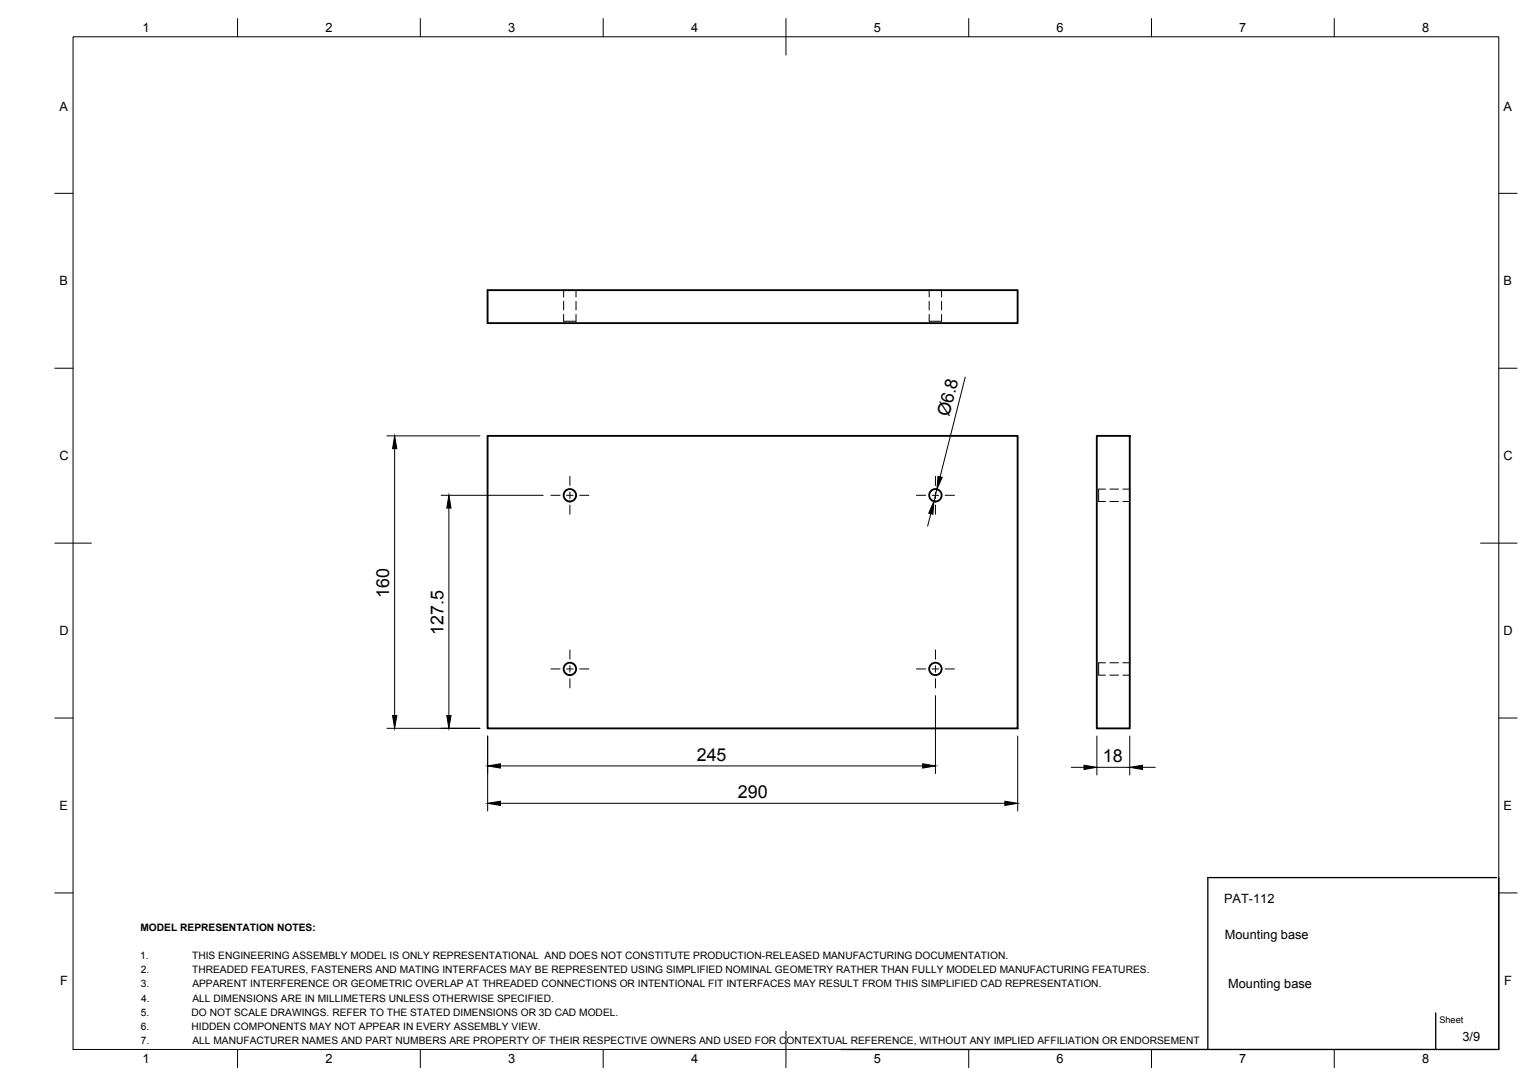
ISO-10303-21;
HEADER;
/* Generated by software containing ST-Developer
 * from STEP Tools, Inc. (www.steptools.com) 
 */

FILE_DESCRIPTION(
/* description */ ('PAT-112'),
/* implementation_level */ '2;1');

FILE_NAME(
/* name */ 'Mounting base.step',
/* time_stamp */ '2026-11-15T15:25:42-08:00',
/* author */ (''),
/* organization */ (''),
/* preprocessor_version */ 'ST-DEVELOPER v20.2',
/* originating_system */ 'Autodesk Translation Framework v15.17.0.0',
/* authorisation */ '');

FILE_SCHEMA (('AUTOMOTIVE_DESIGN { 1 0 10303 214 3 1 1 }'));
ENDSEC;

DATA;
#10=MECHANICAL_DESIGN_GEOMETRIC_PRESENTATION_REPRESENTATION('',(#105),#2277);
#91=SHAPE_REPRESENTATION_RELATIONSHIP('SRR','None',#2319,#98);
#98=ADVANCED_BREP_SHAPE_REPRESENTATION('',(#113),#2269);
#105=STYLED_ITEM('',(#2368),#113);
#113=MANIFOLD_SOLID_BREP('Body1',#1257);
#120=FACE_BOUND('',#287,.T.);
#121=FACE_BOUND('',#288,.T.);
#122=FACE_BOUND('',#289,.T.);
#123=FACE_BOUND('',#290,.T.);
#146=PLANE('',#1349);
#147=PLANE('',#1353);
#148=PLANE('',#1357);
#149=PLANE('',#1361);
#150=PLANE('',#1362);
#151=PLANE('',#1363);
#152=PLANE('',#1364);
#153=PLANE('',#1365);
#154=PLANE('',#1366);
#155=PLANE('',#1367);
#197=FACE_OUTER_BOUND('',#274,.T.);
#198=FACE_OUTER_BOUND('',#275,.T.);
#199=FACE_OUTER_BOUND('',#276,.T.);
#200=FACE_OUTER_BOUND('',#277,.T.);
#201=FACE_OUTER_BOUND('',#278,.T.);
#202=FACE_OUTER_BOUND('',#279,.T.);
#203=FACE_OUTER_BOUND('',#280,.T.);
#204=FACE_OUTER_BOUND('',#281,.T.);
#205=FACE_OUTER_BOUND('',#282,.T.);
#206=FACE_OUTER_BOUND('',#283,.T.);
#207=FACE_OUTER_BOUND('',#284,.T.);
#208=FACE_OUTER_BOUND('',#285,.T.);
#209=FACE_OUTER_BOUND('',#286,.T.);
#210=FACE_OUTER_BOUND('',#291,.T.);
#274=EDGE_LOOP('',(#866,#867,#868,#869));
#275=EDGE_LOOP('',(#870));
#276=EDGE_LOOP('',(#871,#872,#873,#874));
#277=EDGE_LOOP('',(#875));
#278=EDGE_LOOP('',(#876,#877,#878,#879));
#279=EDGE_LOOP('',(#880));
#280=EDGE_LOOP('',(#881,#882,#883,#884));
#281=EDGE_LOOP('',(#885));
#282=EDGE_LOOP('',(#886,#887,#888,#889));
#283=EDGE_LOOP('',(#890,#891,#892,#893));
#284=EDGE_LOOP('',(#894,#895,#896,#897));
#285=EDGE_LOOP('',(#898,#899,#900,#901));
#286=EDGE_LOOP('',(#902,#903,#904,#905));
#287=EDGE_LOOP('',(#906));
#288=EDGE_LOOP('',(#907));
#289=EDGE_LOOP('',(#908));
#290=EDGE_LOOP('',(#909));
#291=EDGE_LOOP('',(#910,#911,#912,#913));
#377=LINE('',#1913,#472);
#378=LINE('',#1920,#473);
#379=LINE('',#1927,#474);
#380=LINE('',#1934,#475);
#381=LINE('',#1940,#476);
#382=LINE('',#1942,#477);
#383=LINE('',#1944,#478);
#384=LINE('',#1945,#479);
#385=LINE('',#1948,#480);
#386=LINE('',#1950,#481);
#387=LINE('',#1951,#482);
#388=LINE('',#1954,#483);
#389=LINE('',#1956,#484);
#390=LINE('',#1957,#485);
#391=LINE('',#1959,#486);
#392=LINE('',#1960,#487);
#472=VECTOR('',#1508,0.34);
#473=VECTOR('',#1517,0.34);
#474=VECTOR('',#1526,0.34);
#475=VECTOR('',#1535,0.34);
#476=VECTOR('',#1542,1.);
#477=VECTOR('',#1543,1.);
#478=VECTOR('',#1544,1.);
#479=VECTOR('',#1545,1.);
#480=VECTOR('',#1548,1.);
#481=VECTOR('',#1549,1.);
#482=VECTOR('',#1550,1.);
#483=VECTOR('',#1553,1.);
#484=VECTOR('',#1554,1.);
#485=VECTOR('',#1555,1.);
#486=VECTOR('',#1558,1.);
#487=VECTOR('',#1559,1.);
#567=CIRCLE('',#1347,0.34);
#568=CIRCLE('',#1348,0.34);
#569=CIRCLE('',#1351,0.34);
#570=CIRCLE('',#1352,0.34);
#571=CIRCLE('',#1355,0.34);
#572=CIRCLE('',#1356,0.34);
#573=CIRCLE('',#1359,0.34);
#574=CIRCLE('',#1360,0.34);
#619=VERTEX_POINT('',#1910);
#620=VERTEX_POINT('',#1912);
#621=VERTEX_POINT('',#1917);
#622=VERTEX_POINT('',#1919);
#623=VERTEX_POINT('',#1924);
#624=VERTEX_POINT('',#1926);
#625=VERTEX_POINT('',#1931);
#626=VERTEX_POINT('',#1933);
#627=VERTEX_POINT('',#1938);
#628=VERTEX_POINT('',#1939);
#629=VERTEX_POINT('',#1941);
#630=VERTEX_POINT('',#1943);
#631=VERTEX_POINT('',#1947);
#632=VERTEX_POINT('',#1949);
#633=VERTEX_POINT('',#1953);
#634=VERTEX_POINT('',#1955);
#719=EDGE_CURVE('',#619,#619,#567,.T.);
#720=EDGE_CURVE('',#619,#620,#377,.T.);
#721=EDGE_CURVE('',#620,#620,#568,.T.);
#722=EDGE_CURVE('',#621,#621,#569,.T.);
#723=EDGE_CURVE('',#621,#622,#378,.T.);
#724=EDGE_CURVE('',#622,#622,#570,.T.);
#725=EDGE_CURVE('',#623,#623,#571,.T.);
#726=EDGE_CURVE('',#623,#624,#379,.T.);
#727=EDGE_CURVE('',#624,#624,#572,.T.);
#728=EDGE_CURVE('',#625,#625,#573,.T.);
#729=EDGE_CURVE('',#625,#626,#380,.T.);
#730=EDGE_CURVE('',#626,#626,#574,.T.);
#731=EDGE_CURVE('',#627,#628,#381,.T.);
#732=EDGE_CURVE('',#628,#629,#382,.T.);
#733=EDGE_CURVE('',#630,#629,#383,.T.);
#734=EDGE_CURVE('',#627,#630,#384,.T.);
#735=EDGE_CURVE('',#631,#627,#385,.T.);
#736=EDGE_CURVE('',#632,#630,#386,.T.);
#737=EDGE_CURVE('',#631,#632,#387,.T.);
#738=EDGE_CURVE('',#633,#631,#388,.T.);
#739=EDGE_CURVE('',#634,#632,#389,.T.);
#740=EDGE_CURVE('',#633,#634,#390,.T.);
#741=EDGE_CURVE('',#628,#633,#391,.T.);
#742=EDGE_CURVE('',#629,#634,#392,.T.);
#866=ORIENTED_EDGE('',*,*,#719,.F.);
#867=ORIENTED_EDGE('',*,*,#720,.T.);
#868=ORIENTED_EDGE('',*,*,#721,.F.);
#869=ORIENTED_EDGE('',*,*,#720,.F.);
#870=ORIENTED_EDGE('',*,*,#719,.T.);
#871=ORIENTED_EDGE('',*,*,#722,.F.);
#872=ORIENTED_EDGE('',*,*,#723,.T.);
#873=ORIENTED_EDGE('',*,*,#724,.F.);
#874=ORIENTED_EDGE('',*,*,#723,.F.);
#875=ORIENTED_EDGE('',*,*,#722,.T.);
#876=ORIENTED_EDGE('',*,*,#725,.F.);
#877=ORIENTED_EDGE('',*,*,#726,.T.);
#878=ORIENTED_EDGE('',*,*,#727,.F.);
#879=ORIENTED_EDGE('',*,*,#726,.F.);
#880=ORIENTED_EDGE('',*,*,#725,.T.);
#881=ORIENTED_EDGE('',*,*,#728,.F.);
#882=ORIENTED_EDGE('',*,*,#729,.T.);
#883=ORIENTED_EDGE('',*,*,#730,.F.);
#884=ORIENTED_EDGE('',*,*,#729,.F.);
#885=ORIENTED_EDGE('',*,*,#728,.T.);
#886=ORIENTED_EDGE('',*,*,#731,.T.);
#887=ORIENTED_EDGE('',*,*,#732,.T.);
#888=ORIENTED_EDGE('',*,*,#733,.F.);
#889=ORIENTED_EDGE('',*,*,#734,.F.);
#890=ORIENTED_EDGE('',*,*,#735,.T.);
#891=ORIENTED_EDGE('',*,*,#734,.T.);
#892=ORIENTED_EDGE('',*,*,#736,.F.);
#893=ORIENTED_EDGE('',*,*,#737,.F.);
#894=ORIENTED_EDGE('',*,*,#738,.T.);
#895=ORIENTED_EDGE('',*,*,#737,.T.);
#896=ORIENTED_EDGE('',*,*,#739,.F.);
#897=ORIENTED_EDGE('',*,*,#740,.F.);
#898=ORIENTED_EDGE('',*,*,#741,.T.);
#899=ORIENTED_EDGE('',*,*,#740,.T.);
#900=ORIENTED_EDGE('',*,*,#742,.F.);
#901=ORIENTED_EDGE('',*,*,#732,.F.);
#902=ORIENTED_EDGE('',*,*,#742,.T.);
#903=ORIENTED_EDGE('',*,*,#739,.T.);
#904=ORIENTED_EDGE('',*,*,#736,.T.);
#905=ORIENTED_EDGE('',*,*,#733,.T.);
#906=ORIENTED_EDGE('',*,*,#721,.T.);
#907=ORIENTED_EDGE('',*,*,#724,.T.);
#908=ORIENTED_EDGE('',*,*,#727,.T.);
#909=ORIENTED_EDGE('',*,*,#730,.T.);
#910=ORIENTED_EDGE('',*,*,#741,.F.);
#911=ORIENTED_EDGE('',*,*,#731,.F.);
#912=ORIENTED_EDGE('',*,*,#735,.F.);
#913=ORIENTED_EDGE('',*,*,#738,.F.);
#1160=CYLINDRICAL_SURFACE('',#1346,0.34);
#1161=CYLINDRICAL_SURFACE('',#1350,0.34);
#1162=CYLINDRICAL_SURFACE('',#1354,0.34);
#1163=CYLINDRICAL_SURFACE('',#1358,0.34);
#1180=ADVANCED_FACE('',(#197),#1160,.F.);
#1181=ADVANCED_FACE('',(#198),#146,.T.);
#1182=ADVANCED_FACE('',(#199),#1161,.F.);
#1183=ADVANCED_FACE('',(#200),#147,.T.);
#1184=ADVANCED_FACE('',(#201),#1162,.F.);
#1185=ADVANCED_FACE('',(#202),#148,.T.);
#1186=ADVANCED_FACE('',(#203),#1163,.F.);
#1187=ADVANCED_FACE('',(#204),#149,.T.);
#1188=ADVANCED_FACE('',(#205),#150,.T.);
#1189=ADVANCED_FACE('',(#206),#151,.T.);
#1190=ADVANCED_FACE('',(#207),#152,.T.);
#1191=ADVANCED_FACE('',(#208),#153,.T.);
#1192=ADVANCED_FACE('',(#209,#120,#121,#122,#123),#154,.T.);
#1193=ADVANCED_FACE('',(#210),#155,.F.);
#1257=CLOSED_SHELL('',(#1180,#1181,#1182,#1183,#1184,#1185,#1186,#1187,
#1188,#1189,#1190,#1191,#1192,#1193));
#1345=AXIS2_PLACEMENT_3D('',#1908,#1502,#1503);
#1346=AXIS2_PLACEMENT_3D('',#1909,#1504,#1505);
#1347=AXIS2_PLACEMENT_3D('',#1911,#1506,#1507);
#1348=AXIS2_PLACEMENT_3D('',#1914,#1509,#1510);
#1349=AXIS2_PLACEMENT_3D('',#1915,#1511,#1512);
#1350=AXIS2_PLACEMENT_3D('',#1916,#1513,#1514);
#1351=AXIS2_PLACEMENT_3D('',#1918,#1515,#1516);
#1352=AXIS2_PLACEMENT_3D('',#1921,#1518,#1519);
#1353=AXIS2_PLACEMENT_3D('',#1922,#1520,#1521);
#1354=AXIS2_PLACEMENT_3D('',#1923,#1522,#1523);
#1355=AXIS2_PLACEMENT_3D('',#1925,#1524,#1525);
#1356=AXIS2_PLACEMENT_3D('',#1928,#1527,#1528);
#1357=AXIS2_PLACEMENT_3D('',#1929,#1529,#1530);
#1358=AXIS2_PLACEMENT_3D('',#1930,#1531,#1532);
#1359=AXIS2_PLACEMENT_3D('',#1932,#1533,#1534);
#1360=AXIS2_PLACEMENT_3D('',#1935,#1536,#1537);
#1361=AXIS2_PLACEMENT_3D('',#1936,#1538,#1539);
#1362=AXIS2_PLACEMENT_3D('',#1937,#1540,#1541);
#1363=AXIS2_PLACEMENT_3D('',#1946,#1546,#1547);
#1364=AXIS2_PLACEMENT_3D('',#1952,#1551,#1552);
#1365=AXIS2_PLACEMENT_3D('',#1958,#1556,#1557);
#1366=AXIS2_PLACEMENT_3D('',#1961,#1560,#1561);
#1367=AXIS2_PLACEMENT_3D('',#1962,#1562,#1563);
#1502=DIRECTION('axis',(0.,0.,1.));
#1503=DIRECTION('refdir',(1.,0.,0.));
#1504=DIRECTION('center_axis',(0.,0.,1.));
#1505=DIRECTION('ref_axis',(1.,0.,0.));
#1506=DIRECTION('center_axis',(0.,0.,1.));
#1507=DIRECTION('ref_axis',(1.,0.,0.));
#1508=DIRECTION('',(0.,0.,1.));
#1509=DIRECTION('center_axis',(0.,0.,-1.));
#1510=DIRECTION('ref_axis',(1.,0.,0.));
#1511=DIRECTION('center_axis',(0.,0.,1.));
#1512=DIRECTION('ref_axis',(1.,0.,0.));
#1513=DIRECTION('center_axis',(0.,0.,1.));
#1514=DIRECTION('ref_axis',(1.,0.,0.));
#1515=DIRECTION('center_axis',(0.,0.,1.));
#1516=DIRECTION('ref_axis',(1.,0.,0.));
#1517=DIRECTION('',(0.,0.,1.));
#1518=DIRECTION('center_axis',(0.,0.,-1.));
#1519=DIRECTION('ref_axis',(1.,0.,0.));
#1520=DIRECTION('center_axis',(0.,0.,1.));
#1521=DIRECTION('ref_axis',(1.,0.,0.));
#1522=DIRECTION('center_axis',(0.,0.,1.));
#1523=DIRECTION('ref_axis',(1.,0.,0.));
#1524=DIRECTION('center_axis',(0.,0.,1.));
#1525=DIRECTION('ref_axis',(1.,0.,0.));
#1526=DIRECTION('',(0.,0.,1.));
#1527=DIRECTION('center_axis',(0.,0.,-1.));
#1528=DIRECTION('ref_axis',(1.,0.,0.));
#1529=DIRECTION('center_axis',(0.,0.,1.));
#1530=DIRECTION('ref_axis',(1.,0.,0.));
#1531=DIRECTION('center_axis',(0.,0.,1.));
#1532=DIRECTION('ref_axis',(1.,0.,0.));
#1533=DIRECTION('center_axis',(0.,0.,1.));
#1534=DIRECTION('ref_axis',(1.,0.,0.));
#1535=DIRECTION('',(0.,0.,1.));
#1536=DIRECTION('center_axis',(0.,0.,-1.));
#1537=DIRECTION('ref_axis',(1.,0.,0.));
#1538=DIRECTION('center_axis',(0.,0.,1.));
#1539=DIRECTION('ref_axis',(1.,0.,0.));
#1540=DIRECTION('center_axis',(0.,1.,0.));
#1541=DIRECTION('ref_axis',(-1.,0.,0.));
#1542=DIRECTION('',(-1.,0.,0.));
#1543=DIRECTION('',(0.,0.,1.));
#1544=DIRECTION('',(-1.,0.,0.));
#1545=DIRECTION('',(0.,0.,1.));
#1546=DIRECTION('center_axis',(1.,0.,0.));
#1547=DIRECTION('ref_axis',(0.,1.,0.));
#1548=DIRECTION('',(0.,1.,0.));
#1549=DIRECTION('',(0.,1.,0.));
#1550=DIRECTION('',(0.,0.,1.));
#1551=DIRECTION('center_axis',(0.,-1.,0.));
#1552=DIRECTION('ref_axis',(1.,0.,0.));
#1553=DIRECTION('',(1.,0.,0.));
#1554=DIRECTION('',(1.,0.,0.));
#1555=DIRECTION('',(0.,0.,1.));
#1556=DIRECTION('center_axis',(-1.,0.,0.));
#1557=DIRECTION('ref_axis',(0.,-1.,0.));
#1558=DIRECTION('',(0.,-1.,0.));
#1559=DIRECTION('',(0.,-1.,0.));
#1560=DIRECTION('center_axis',(0.,0.,1.));
#1561=DIRECTION('ref_axis',(1.,0.,0.));
#1562=DIRECTION('center_axis',(0.,0.,1.));
#1563=DIRECTION('ref_axis',(1.,0.,0.));
#1908=CARTESIAN_POINT('',(0.,0.,0.));
#1909=CARTESIAN_POINT('Origin',(4.75,20.,-0.5));
#1910=CARTESIAN_POINT('',(4.41,20.,-0.5));
#1911=CARTESIAN_POINT('Origin',(4.75,20.,-0.5));
#1912=CARTESIAN_POINT('',(4.41,20.,1.2));
#1913=CARTESIAN_POINT('',(4.41,20.,-0.5));
#1914=CARTESIAN_POINT('Origin',(4.75,20.,1.2));
#1915=CARTESIAN_POINT('Origin',(4.75,20.,-0.5));
#1916=CARTESIAN_POINT('Origin',(-4.75,20.,-0.5));
#1917=CARTESIAN_POINT('',(-5.09,20.,-0.5));
#1918=CARTESIAN_POINT('Origin',(-4.75,20.,-0.5));
#1919=CARTESIAN_POINT('',(-5.09,20.,1.2));
#1920=CARTESIAN_POINT('',(-5.09,20.,-0.5));
#1921=CARTESIAN_POINT('Origin',(-4.75,20.,1.2));
#1922=CARTESIAN_POINT('Origin',(-4.75,20.,-0.5));
#1923=CARTESIAN_POINT('Origin',(4.75,0.,-0.5));
#1924=CARTESIAN_POINT('',(4.41,-4.163799117101E-17,-0.5));
#1925=CARTESIAN_POINT('Origin',(4.75,0.,-0.5));
#1926=CARTESIAN_POINT('',(4.41,4.163799117101E-17,1.2));
#1927=CARTESIAN_POINT('',(4.41,-4.163799117101E-17,-0.5));
#1928=CARTESIAN_POINT('Origin',(4.75,0.,1.2));
#1929=CARTESIAN_POINT('Origin',(4.75,0.,-0.5));
#1930=CARTESIAN_POINT('Origin',(-4.75,0.,-0.5));
#1931=CARTESIAN_POINT('',(-5.09,-4.163799117101E-17,-0.5));
#1932=CARTESIAN_POINT('Origin',(-4.75,0.,-0.5));
#1933=CARTESIAN_POINT('',(-5.09,4.163799117101E-17,1.2));
#1934=CARTESIAN_POINT('',(-5.09,-4.163799117101E-17,-0.5));
#1935=CARTESIAN_POINT('Origin',(-4.75,0.,1.2));
#1936=CARTESIAN_POINT('Origin',(-4.75,0.,-0.5));
#1937=CARTESIAN_POINT('Origin',(8.,24.5,-0.6));
#1938=CARTESIAN_POINT('',(8.,24.5,-0.6));
#1939=CARTESIAN_POINT('',(-8.,24.5,-0.6));
#1940=CARTESIAN_POINT('',(8.,24.5,-0.6));
#1941=CARTESIAN_POINT('',(-8.,24.5,1.2));
#1942=CARTESIAN_POINT('',(-8.,24.5,-0.6));
#1943=CARTESIAN_POINT('',(8.,24.5,1.2));
#1944=CARTESIAN_POINT('',(8.,24.5,1.2));
#1945=CARTESIAN_POINT('',(8.,24.5,-0.6));
#1946=CARTESIAN_POINT('Origin',(8.,-4.5,-0.6));
#1947=CARTESIAN_POINT('',(8.,-4.5,-0.6));
#1948=CARTESIAN_POINT('',(8.,-4.5,-0.6));
#1949=CARTESIAN_POINT('',(8.,-4.5,1.2));
#1950=CARTESIAN_POINT('',(8.,-4.5,1.2));
#1951=CARTESIAN_POINT('',(8.,-4.5,-0.6));
#1952=CARTESIAN_POINT('Origin',(-8.,-4.5,-0.6));
#1953=CARTESIAN_POINT('',(-8.,-4.5,-0.6));
#1954=CARTESIAN_POINT('',(-8.,-4.5,-0.6));
#1955=CARTESIAN_POINT('',(-8.,-4.5,1.2));
#1956=CARTESIAN_POINT('',(-8.,-4.5,1.2));
#1957=CARTESIAN_POINT('',(-8.,-4.5,-0.6));
#1958=CARTESIAN_POINT('Origin',(-8.,24.5,-0.6));
#1959=CARTESIAN_POINT('',(-8.,24.5,-0.6));
#1960=CARTESIAN_POINT('',(-8.,24.5,1.2));
#1961=CARTESIAN_POINT('Origin',(0.,10.,1.2));
#1962=CARTESIAN_POINT('Origin',(0.,10.,-0.6));
#2259=UNCERTAINTY_MEASURE_WITH_UNIT(LENGTH_MEASURE(0.001),#2278,
'DISTANCE_ACCURACY_VALUE',
'Maximum model space distance between geometric entities at asserted c
onnectivities');
#2267=UNCERTAINTY_MEASURE_WITH_UNIT(LENGTH_MEASURE(0.001),#2278,
'DISTANCE_ACCURACY_VALUE',
'Maximum model space distance between geometric entities at asserted c
onnectivities');
#2269=(
GEOMETRIC_REPRESENTATION_CONTEXT(3)
GLOBAL_UNCERTAINTY_ASSIGNED_CONTEXT((#2259))
GLOBAL_UNIT_ASSIGNED_CONTEXT((#2278,#2280,#2281))
REPRESENTATION_CONTEXT('','3D')
);
#2277=(
GEOMETRIC_REPRESENTATION_CONTEXT(3)
GLOBAL_UNCERTAINTY_ASSIGNED_CONTEXT((#2267))
GLOBAL_UNIT_ASSIGNED_CONTEXT((#2278,#2280,#2281))
REPRESENTATION_CONTEXT('','3D')
);
#2278=(
LENGTH_UNIT()
NAMED_UNIT(*)
SI_UNIT(.CENTI.,.METRE.)
);
#2280=(
NAMED_UNIT(*)
PLANE_ANGLE_UNIT()
SI_UNIT($,.RADIAN.)
);
#2281=(
NAMED_UNIT(*)
SI_UNIT($,.STERADIAN.)
SOLID_ANGLE_UNIT()
);
#2283=SHAPE_DEFINITION_REPRESENTATION(#2292,#2319);
#2292=PRODUCT_DEFINITION_SHAPE('',$,#2329);
#2319=SHAPE_REPRESENTATION('',(#1345),#2269);
#2327=PRODUCT_DEFINITION_CONTEXT('part definition',#2356,'design');
#2329=PRODUCT_DEFINITION('Mounting base','Mounting base',#2338,#2327);
#2338=PRODUCT_DEFINITION_FORMATION('',$,#2359);
#2356=APPLICATION_CONTEXT(
'Core Data for Automotive Mechanical Design Process');
#2357=PRODUCT_CONTEXT('part definition',#2356,'mechanical');
#2359=PRODUCT('Mounting base','Mounting base','Mounting base',(#2357));
#2368=PRESENTATION_STYLE_ASSIGNMENT((#2373));
#2373=SURFACE_STYLE_USAGE(.BOTH.,#2378);
#2378=SURFACE_SIDE_STYLE('',(#2383));
#2383=SURFACE_STYLE_FILL_AREA(#2388);
#2388=FILL_AREA_STYLE('Opaque(20,51,87)',(#2393));
#2393=FILL_AREA_STYLE_COLOUR('Opaque(20,51,87)',#2398);
#2398=COLOUR_RGB('Opaque(20,51,87)',0.0784313725490196,0.2,0.341176470588235);
ENDSEC;
END-ISO-10303-21;
